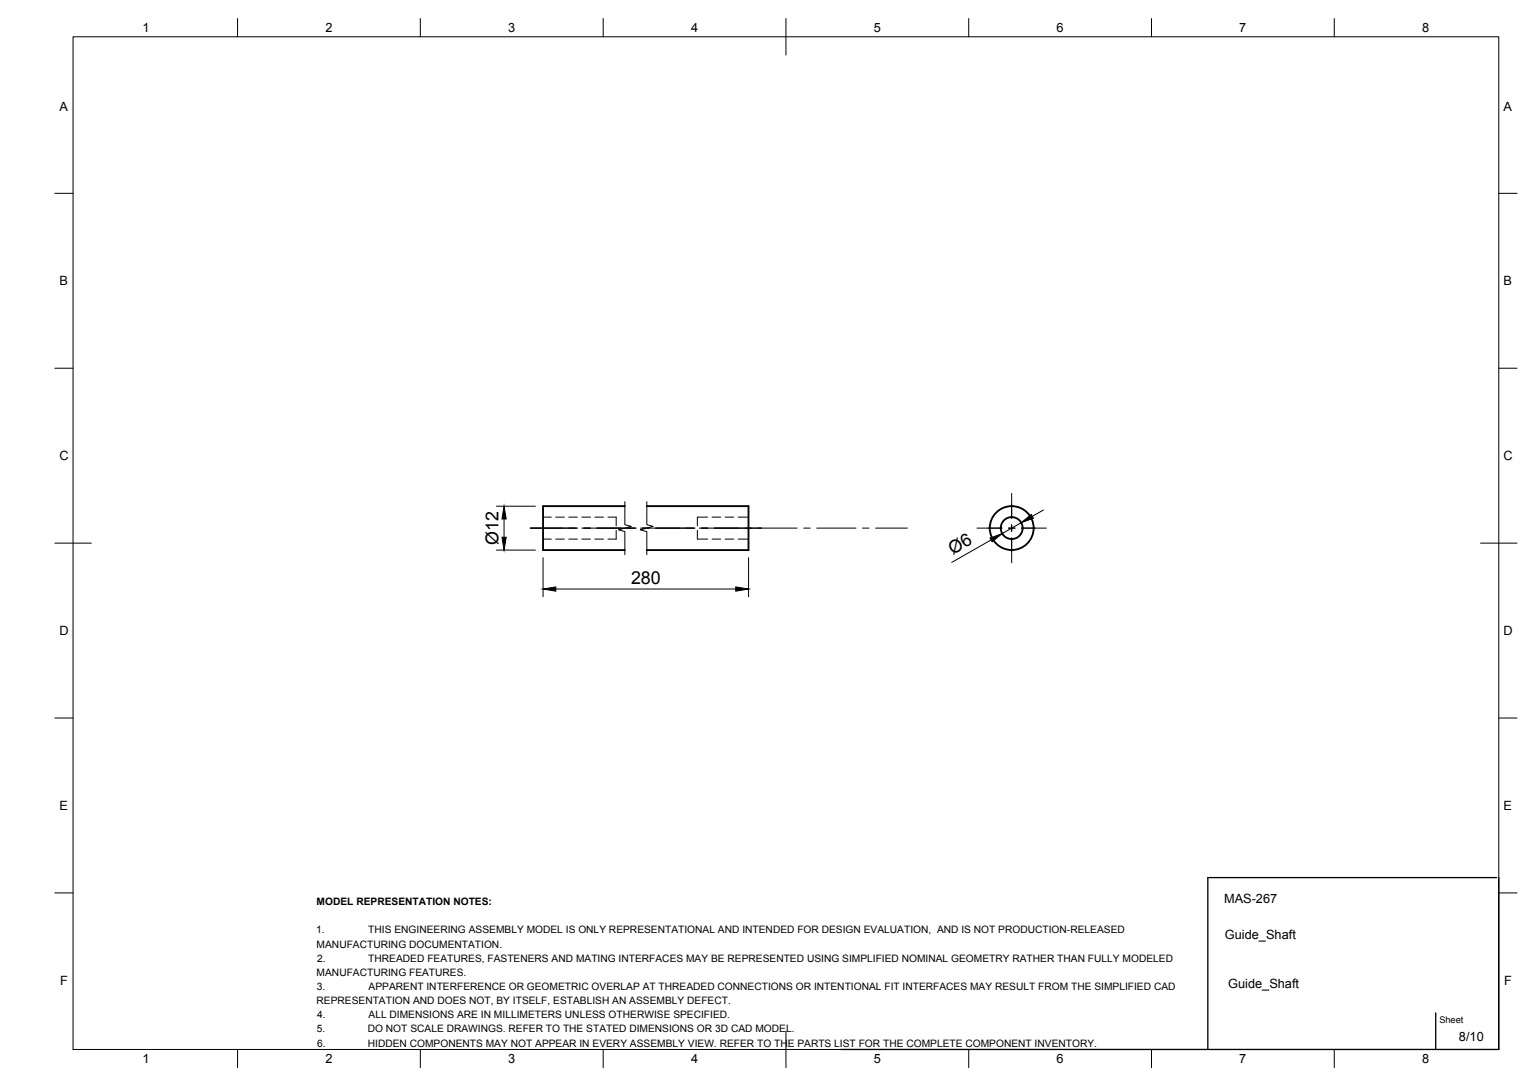
ISO-10303-21;
HEADER;
/* Generated by software containing ST-Developer
 * from STEP Tools, Inc. (www.steptools.com) 
 */

FILE_DESCRIPTION(
/* description */ (''),
/* implementation_level */ '2;1');

FILE_NAME(
/* name */ 'Guide_Shaft.step',
/* time_stamp */ '2026-10-12T15:29:24-07:00',
/* author */ (''),
/* organization */ (''),
/* preprocessor_version */ 'ST-DEVELOPER v20.2',
/* originating_system */ 'Autodesk Translation Framework v15.15.0.0',
/* authorisation */ '');

FILE_SCHEMA (('AUTOMOTIVE_DESIGN { 1 0 10303 214 3 1 1 }'));
ENDSEC;

DATA;
#10=MECHANICAL_DESIGN_GEOMETRIC_PRESENTATION_REPRESENTATION('',(#197),#9496);
#151=SHAPE_REPRESENTATION_RELATIONSHIP('SRR','None',#9545,#160);
#160=ADVANCED_BREP_SHAPE_REPRESENTATION('',(#254),#9493);
#197=STYLED_ITEM('',(#9594),#254);
#254=MANIFOLD_SOLID_BREP('Body1',#4999);
#416=FACE_BOUND('',#1254,.T.);
#417=FACE_BOUND('',#1257,.T.);
#566=PLANE('',#5566);
#567=PLANE('',#5570);
#568=PLANE('',#5571);
#569=PLANE('',#5575);
#834=FACE_OUTER_BOUND('',#1249,.T.);
#835=FACE_OUTER_BOUND('',#1250,.T.);
#836=FACE_OUTER_BOUND('',#1251,.T.);
#837=FACE_OUTER_BOUND('',#1252,.T.);
#838=FACE_OUTER_BOUND('',#1253,.T.);
#839=FACE_OUTER_BOUND('',#1255,.T.);
#840=FACE_OUTER_BOUND('',#1256,.T.);
#1249=EDGE_LOOP('',(#4053,#4054,#4055,#4056));
#1250=EDGE_LOOP('',(#4057));
#1251=EDGE_LOOP('',(#4058,#4059,#4060,#4061));
#1252=EDGE_LOOP('',(#4062));
#1253=EDGE_LOOP('',(#4063));
#1254=EDGE_LOOP('',(#4064));
#1255=EDGE_LOOP('',(#4065,#4066,#4067,#4068));
#1256=EDGE_LOOP('',(#4069));
#1257=EDGE_LOOP('',(#4070));
#1566=LINE('',#8632,#1803);
#1567=LINE('',#8639,#1804);
#1568=LINE('',#8648,#1805);
#1803=VECTOR('',#6843,3.);
#1804=VECTOR('',#6852,3.);
#1805=VECTOR('',#6865,6.00000000000001);
#2140=CIRCLE('',#5564,3.);
#2141=CIRCLE('',#5565,3.);
#2142=CIRCLE('',#5568,3.);
#2143=CIRCLE('',#5569,3.);
#2144=CIRCLE('',#5572,6.00000000000001);
#2145=CIRCLE('',#5574,6.00000000000001);
#2525=VERTEX_POINT('',#8629);
#2526=VERTEX_POINT('',#8631);
#2527=VERTEX_POINT('',#8636);
#2528=VERTEX_POINT('',#8638);
#2529=VERTEX_POINT('',#8643);
#2530=VERTEX_POINT('',#8646);
#3079=EDGE_CURVE('',#2525,#2525,#2140,.T.);
#3080=EDGE_CURVE('',#2525,#2526,#1566,.T.);
#3081=EDGE_CURVE('',#2526,#2526,#2141,.T.);
#3082=EDGE_CURVE('',#2527,#2527,#2142,.T.);
#3083=EDGE_CURVE('',#2527,#2528,#1567,.T.);
#3084=EDGE_CURVE('',#2528,#2528,#2143,.T.);
#3085=EDGE_CURVE('',#2529,#2529,#2144,.T.);
#3086=EDGE_CURVE('',#2530,#2530,#2145,.T.);
#3087=EDGE_CURVE('',#2530,#2529,#1568,.T.);
#4053=ORIENTED_EDGE('',*,*,#3079,.F.);
#4054=ORIENTED_EDGE('',*,*,#3080,.T.);
#4055=ORIENTED_EDGE('',*,*,#3081,.T.);
#4056=ORIENTED_EDGE('',*,*,#3080,.F.);
#4057=ORIENTED_EDGE('',*,*,#3081,.F.);
#4058=ORIENTED_EDGE('',*,*,#3082,.F.);
#4059=ORIENTED_EDGE('',*,*,#3083,.T.);
#4060=ORIENTED_EDGE('',*,*,#3084,.T.);
#4061=ORIENTED_EDGE('',*,*,#3083,.F.);
#4062=ORIENTED_EDGE('',*,*,#3084,.F.);
#4063=ORIENTED_EDGE('',*,*,#3085,.T.);
#4064=ORIENTED_EDGE('',*,*,#3079,.T.);
#4065=ORIENTED_EDGE('',*,*,#3086,.F.);
#4066=ORIENTED_EDGE('',*,*,#3087,.T.);
#4067=ORIENTED_EDGE('',*,*,#3085,.F.);
#4068=ORIENTED_EDGE('',*,*,#3087,.F.);
#4069=ORIENTED_EDGE('',*,*,#3086,.T.);
#4070=ORIENTED_EDGE('',*,*,#3082,.T.);
#4607=CYLINDRICAL_SURFACE('',#5563,3.);
#4608=CYLINDRICAL_SURFACE('',#5567,3.);
#4609=CYLINDRICAL_SURFACE('',#5573,6.00000000000001);
#4845=ADVANCED_FACE('',(#834),#4607,.F.);
#4846=ADVANCED_FACE('',(#835),#566,.T.);
#4847=ADVANCED_FACE('',(#836),#4608,.F.);
#4848=ADVANCED_FACE('',(#837),#567,.T.);
#4849=ADVANCED_FACE('',(#838,#416),#568,.F.);
#4850=ADVANCED_FACE('',(#839),#4609,.T.);
#4851=ADVANCED_FACE('',(#840,#417),#569,.T.);
#4999=CLOSED_SHELL('',(#4845,#4846,#4847,#4848,#4849,#4850,#4851));
#5562=AXIS2_PLACEMENT_3D('',#8627,#6837,#6838);
#5563=AXIS2_PLACEMENT_3D('',#8628,#6839,#6840);
#5564=AXIS2_PLACEMENT_3D('',#8630,#6841,#6842);
#5565=AXIS2_PLACEMENT_3D('',#8633,#6844,#6845);
#5566=AXIS2_PLACEMENT_3D('',#8634,#6846,#6847);
#5567=AXIS2_PLACEMENT_3D('',#8635,#6848,#6849);
#5568=AXIS2_PLACEMENT_3D('',#8637,#6850,#6851);
#5569=AXIS2_PLACEMENT_3D('',#8640,#6853,#6854);
#5570=AXIS2_PLACEMENT_3D('',#8641,#6855,#6856);
#5571=AXIS2_PLACEMENT_3D('',#8642,#6857,#6858);
#5572=AXIS2_PLACEMENT_3D('',#8644,#6859,#6860);
#5573=AXIS2_PLACEMENT_3D('',#8645,#6861,#6862);
#5574=AXIS2_PLACEMENT_3D('',#8647,#6863,#6864);
#5575=AXIS2_PLACEMENT_3D('',#8649,#6866,#6867);
#6837=DIRECTION('axis',(0.,0.,1.));
#6838=DIRECTION('refdir',(1.,0.,0.));
#6839=DIRECTION('center_axis',(1.,0.,0.));
#6840=DIRECTION('ref_axis',(0.,-1.,0.));
#6841=DIRECTION('center_axis',(1.,0.,0.));
#6842=DIRECTION('ref_axis',(0.,-1.,0.));
#6843=DIRECTION('',(1.,0.,0.));
#6844=DIRECTION('center_axis',(1.,0.,0.));
#6845=DIRECTION('ref_axis',(0.,-1.,0.));
#6846=DIRECTION('center_axis',(-1.,0.,0.));
#6847=DIRECTION('ref_axis',(0.,-1.,0.));
#6848=DIRECTION('center_axis',(-1.,0.,0.));
#6849=DIRECTION('ref_axis',(0.,1.,0.));
#6850=DIRECTION('center_axis',(-1.,0.,0.));
#6851=DIRECTION('ref_axis',(0.,1.,0.));
#6852=DIRECTION('',(-1.,0.,0.));
#6853=DIRECTION('center_axis',(-1.,0.,0.));
#6854=DIRECTION('ref_axis',(0.,1.,0.));
#6855=DIRECTION('center_axis',(1.,0.,0.));
#6856=DIRECTION('ref_axis',(0.,1.,0.));
#6857=DIRECTION('center_axis',(1.,0.,0.));
#6858=DIRECTION('ref_axis',(0.,1.,0.));
#6859=DIRECTION('center_axis',(-1.,0.,0.));
#6860=DIRECTION('ref_axis',(0.,1.,0.));
#6861=DIRECTION('center_axis',(1.,0.,0.));
#6862=DIRECTION('ref_axis',(0.,1.,0.));
#6863=DIRECTION('center_axis',(1.,0.,0.));
#6864=DIRECTION('ref_axis',(0.,1.,0.));
#6865=DIRECTION('',(-1.,0.,0.));
#6866=DIRECTION('center_axis',(1.,0.,0.));
#6867=DIRECTION('ref_axis',(0.,1.,0.));
#8627=CARTESIAN_POINT('',(0.,0.,0.));
#8628=CARTESIAN_POINT('Origin',(-150.,-37.8343839603864,-7.99999999999999));
#8629=CARTESIAN_POINT('',(-140.,-34.8343839603864,-7.99999999999999));
#8630=CARTESIAN_POINT('Origin',(-140.,-37.8343839603864,-7.99999999999999));
#8631=CARTESIAN_POINT('',(-126.,-34.8343839603864,-7.99999999999999));
#8632=CARTESIAN_POINT('',(-150.,-34.8343839603864,-7.99999999999999));
#8633=CARTESIAN_POINT('Origin',(-126.,-37.8343839603864,-7.99999999999999));
#8634=CARTESIAN_POINT('Origin',(-126.,-37.8343839603864,-7.99999999999999));
#8635=CARTESIAN_POINT('Origin',(150.,-37.8343839603864,-8.00000000000001));
#8636=CARTESIAN_POINT('',(140.,-40.8343839603864,-8.00000000000001));
#8637=CARTESIAN_POINT('Origin',(140.,-37.8343839603864,-8.00000000000001));
#8638=CARTESIAN_POINT('',(120.,-40.8343839603864,-8.00000000000001));
#8639=CARTESIAN_POINT('',(150.,-40.8343839603864,-8.00000000000001));
#8640=CARTESIAN_POINT('Origin',(120.,-37.8343839603864,-8.00000000000001));
#8641=CARTESIAN_POINT('Origin',(120.,-37.8343839603864,-8.00000000000001));
#8642=CARTESIAN_POINT('Origin',(-140.,-37.8343839603864,-7.99999999999999));
#8643=CARTESIAN_POINT('',(-140.,-43.8343839603864,-7.99999999999999));
#8644=CARTESIAN_POINT('Origin',(-140.,-37.8343839603864,-7.99999999999999));
#8645=CARTESIAN_POINT('Origin',(0.,-37.8343839603864,-7.99999999999999));
#8646=CARTESIAN_POINT('',(140.,-43.8343839603864,-7.99999999999999));
#8647=CARTESIAN_POINT('Origin',(140.,-37.8343839603864,-7.99999999999999));
#8648=CARTESIAN_POINT('',(0.,-43.8343839603864,-7.99999999999999));
#8649=CARTESIAN_POINT('Origin',(140.,-37.8343839603864,-7.99999999999999));
#9482=UNCERTAINTY_MEASURE_WITH_UNIT(LENGTH_MEASURE(0.01),#9497,
'DISTANCE_ACCURACY_VALUE',
'Maximum model space distance between geometric entities at asserted c
onnectivities');
#9485=UNCERTAINTY_MEASURE_WITH_UNIT(LENGTH_MEASURE(0.01),#9497,
'DISTANCE_ACCURACY_VALUE',
'Maximum model space distance between geometric entities at asserted c
onnectivities');
#9493=(
GEOMETRIC_REPRESENTATION_CONTEXT(3)
GLOBAL_UNCERTAINTY_ASSIGNED_CONTEXT((#9482))
GLOBAL_UNIT_ASSIGNED_CONTEXT((#9497,#9499,#9500))
REPRESENTATION_CONTEXT('','3D')
);
#9496=(
GEOMETRIC_REPRESENTATION_CONTEXT(3)
GLOBAL_UNCERTAINTY_ASSIGNED_CONTEXT((#9485))
GLOBAL_UNIT_ASSIGNED_CONTEXT((#9497,#9499,#9500))
REPRESENTATION_CONTEXT('','3D')
);
#9497=(
LENGTH_UNIT()
NAMED_UNIT(*)
SI_UNIT(.MILLI.,.METRE.)
);
#9499=(
NAMED_UNIT(*)
PLANE_ANGLE_UNIT()
SI_UNIT($,.RADIAN.)
);
#9500=(
NAMED_UNIT(*)
SI_UNIT($,.STERADIAN.)
SOLID_ANGLE_UNIT()
);
#9508=SHAPE_DEFINITION_REPRESENTATION(#9518,#9545);
#9518=PRODUCT_DEFINITION_SHAPE('',$,#9556);
#9545=SHAPE_REPRESENTATION('',(#5562),#9493);
#9548=PRODUCT_DEFINITION_CONTEXT('part definition',#9580,'design');
#9556=PRODUCT_DEFINITION('Guide_Shaft','Guide_Shaft',#9566,#9548);
#9566=PRODUCT_DEFINITION_FORMATION('',$,#9589);
#9580=APPLICATION_CONTEXT(
'Core Data for Automotive Mechanical Design Process');
#9581=PRODUCT_CONTEXT('part definition',#9580,'mechanical');
#9589=PRODUCT('Guide_Shaft','Guide_Shaft',$,(#9581));
#9594=PRESENTATION_STYLE_ASSIGNMENT((#9597));
#9597=SURFACE_STYLE_USAGE(.BOTH.,#9600);
#9600=SURFACE_SIDE_STYLE('',(#9603));
#9603=SURFACE_STYLE_FILL_AREA(#9606);
#9606=FILL_AREA_STYLE('Opaque(160,160,160)',(#9609));
#9609=FILL_AREA_STYLE_COLOUR('Opaque(160,160,160)',#9612);
#9612=COLOUR_RGB('Opaque(160,160,160)', 0.40784314, 0.44705882, 0.49803922);
ENDSEC;
END-ISO-10303-21;
